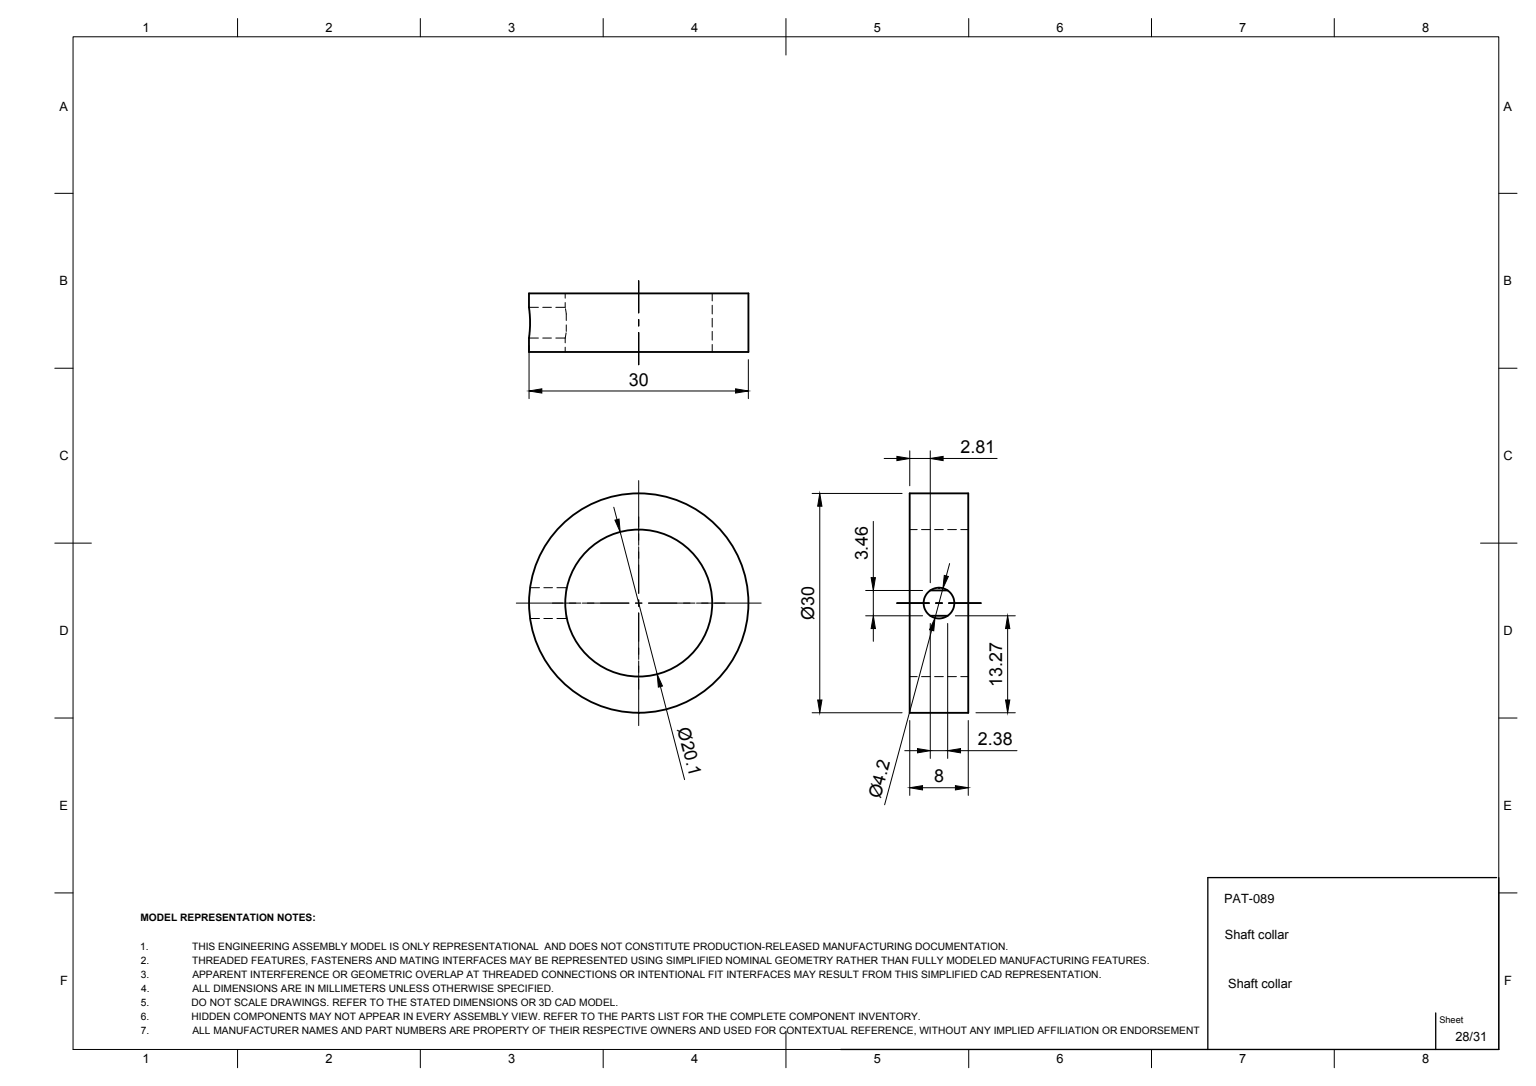
ISO-10303-21;
HEADER;
/* Generated by software containing ST-Developer
 * from STEP Tools, Inc. (www.steptools.com) 
 */

FILE_DESCRIPTION(
/* description */ ('Rotary union on bearing shaft'),
/* implementation_level */ '2;1');

FILE_NAME(
/* name */ 'Shaft collar.step',
/* time_stamp */ '2026-10-28T03:24:01-07:00',
/* author */ (''),
/* organization */ (''),
/* preprocessor_version */ 'ST-DEVELOPER v20.2',
/* originating_system */ 'Autodesk Translation Framework v15.17.0.0',
/* authorisation */ '');

FILE_SCHEMA (('AUTOMOTIVE_DESIGN { 1 0 10303 214 3 1 1 }'));
ENDSEC;

DATA;
#10=MECHANICAL_DESIGN_GEOMETRIC_PRESENTATION_REPRESENTATION('',(#341),#9448);
#255=B_SPLINE_CURVE_WITH_KNOTS('',3,(#8940,#8941,#8942,#8943,#8944,#8945,
#8946,#8947,#8948,#8949,#8950,#8951,#8952,#8953),.UNSPECIFIED.,.F.,.F.,
(4,2,2,2,2,2,4),(0.756005737987012,0.793568827564648,0.872922520054202,
0.952276212543757,1.03162990503331,1.11098359752287,1.1485466871005),
 .UNSPECIFIED.);
#256=B_SPLINE_CURVE_WITH_KNOTS('',3,(#8959,#8960,#8961,#8962,#8963,#8964,
#8965,#8966,#8967,#8968,#8969,#8970,#8971,#8972,#8973,#8974,#8975,#8976),
 .UNSPECIFIED.,.F.,.F.,(4,2,2,2,2,2,2,2,4),(0.,0.0792165807733632,0.158433161546726,
0.237648697074571,0.316864232602415,0.396079768130259,0.475295303658103,
0.554511884431466,0.63372846520483),.UNSPECIFIED.);
#257=B_SPLINE_CURVE_WITH_KNOTS('',3,(#8977,#8978,#8979,#8980,#8981,#8982,
#8983,#8984,#8985,#8986,#8987,#8988,#8989,#8990,#8991,#8992,#8993,#8994),
 .UNSPECIFIED.,.F.,.F.,(4,2,2,2,2,2,2,2,4),(0.63372846520483,0.712945045978192,
0.792161626751555,0.8713771622794,0.950592697807244,1.02980823333509,1.10902376886293,
1.1882403496363,1.26745693040966),.UNSPECIFIED.);
#258=B_SPLINE_CURVE_WITH_KNOTS('',3,(#8997,#8998,#8999,#9000,#9001,#9002,
#9003,#9004,#9005,#9006,#9007,#9008,#9009,#9010),.UNSPECIFIED.,.F.,.F.,
(4,2,2,2,2,2,4),(0.121154929624506,0.158718019202143,0.238071711691698,
0.317425404181252,0.396779096670807,0.476132789160362,0.513695878738),
 .UNSPECIFIED.);
#279=SHAPE_REPRESENTATION_RELATIONSHIP('SRR','None',#9581,#306);
#306=ADVANCED_BREP_SHAPE_REPRESENTATION('',(#374),#9441);
#341=STYLED_ITEM('',(#9778),#374);
#374=MANIFOLD_SOLID_BREP('Body1',#4898);
#464=FACE_BOUND('',#1264,.T.);
#465=FACE_BOUND('',#1266,.T.);
#466=FACE_BOUND('',#1268,.T.);
#467=FACE_BOUND('',#1270,.T.);
#604=PLANE('',#5662);
#605=PLANE('',#5667);
#606=PLANE('',#5674);
#607=PLANE('',#5675);
#877=FACE_OUTER_BOUND('',#1260,.T.);
#878=FACE_OUTER_BOUND('',#1261,.T.);
#879=FACE_OUTER_BOUND('',#1262,.T.);
#880=FACE_OUTER_BOUND('',#1263,.T.);
#881=FACE_OUTER_BOUND('',#1265,.T.);
#882=FACE_OUTER_BOUND('',#1267,.T.);
#883=FACE_OUTER_BOUND('',#1269,.T.);
#1260=EDGE_LOOP('',(#4151,#4152));
#1261=EDGE_LOOP('',(#4153,#4154,#4155,#4156,#4157,#4158,#4159,#4160,#4161));
#1262=EDGE_LOOP('',(#4162,#4163,#4164));
#1263=EDGE_LOOP('',(#4165,#4166,#4167,#4168));
#1264=EDGE_LOOP('',(#4169,#4170,#4171,#4172));
#1265=EDGE_LOOP('',(#4173,#4174,#4175,#4176));
#1266=EDGE_LOOP('',(#4177,#4178));
#1267=EDGE_LOOP('',(#4179));
#1268=EDGE_LOOP('',(#4180));
#1269=EDGE_LOOP('',(#4181));
#1270=EDGE_LOOP('',(#4182));
#1566=LINE('',#8936,#1886);
#1567=LINE('',#8957,#1887);
#1568=LINE('',#9012,#1888);
#1569=LINE('',#9017,#1889);
#1570=LINE('',#9023,#1890);
#1886=VECTOR('',#6951,1.);
#1887=VECTOR('',#6958,0.21);
#1888=VECTOR('',#6963,1.);
#1889=VECTOR('',#6968,1.005);
#1890=VECTOR('',#6975,1.5);
#2208=CIRCLE('',#5663,0.21);
#2209=CIRCLE('',#5665,0.21);
#2210=CIRCLE('',#5666,0.21);
#2211=CIRCLE('',#5669,1.005);
#2212=CIRCLE('',#5670,1.005);
#2213=CIRCLE('',#5672,1.5);
#2214=CIRCLE('',#5673,1.5);
#2554=VERTEX_POINT('',#8934);
#2555=VERTEX_POINT('',#8935);
#2556=VERTEX_POINT('',#8939);
#2557=VERTEX_POINT('',#8954);
#2558=VERTEX_POINT('',#8956);
#2559=VERTEX_POINT('',#8958);
#2560=VERTEX_POINT('',#8995);
#2561=VERTEX_POINT('',#9014);
#2562=VERTEX_POINT('',#9016);
#2563=VERTEX_POINT('',#9020);
#2564=VERTEX_POINT('',#9022);
#3103=EDGE_CURVE('',#2554,#2555,#1566,.T.);
#3104=EDGE_CURVE('',#2554,#2555,#2208,.T.);
#3105=EDGE_CURVE('',#2556,#2554,#255,.T.);
#3106=EDGE_CURVE('',#2557,#2556,#2209,.T.);
#3107=EDGE_CURVE('',#2557,#2558,#1567,.T.);
#3108=EDGE_CURVE('',#2559,#2558,#256,.T.);
#3109=EDGE_CURVE('',#2558,#2559,#257,.T.);
#3110=EDGE_CURVE('',#2560,#2557,#2210,.T.);
#3111=EDGE_CURVE('',#2555,#2560,#258,.T.);
#3112=EDGE_CURVE('',#2560,#2556,#1568,.T.);
#3113=EDGE_CURVE('',#2561,#2561,#2211,.T.);
#3114=EDGE_CURVE('',#2561,#2562,#1569,.T.);
#3115=EDGE_CURVE('',#2562,#2562,#2212,.T.);
#3116=EDGE_CURVE('',#2563,#2563,#2213,.T.);
#3117=EDGE_CURVE('',#2563,#2564,#1570,.T.);
#3118=EDGE_CURVE('',#2564,#2564,#2214,.T.);
#4151=ORIENTED_EDGE('',*,*,#3103,.F.);
#4152=ORIENTED_EDGE('',*,*,#3104,.T.);
#4153=ORIENTED_EDGE('',*,*,#3105,.F.);
#4154=ORIENTED_EDGE('',*,*,#3106,.F.);
#4155=ORIENTED_EDGE('',*,*,#3107,.T.);
#4156=ORIENTED_EDGE('',*,*,#3108,.F.);
#4157=ORIENTED_EDGE('',*,*,#3109,.F.);
#4158=ORIENTED_EDGE('',*,*,#3107,.F.);
#4159=ORIENTED_EDGE('',*,*,#3110,.F.);
#4160=ORIENTED_EDGE('',*,*,#3111,.F.);
#4161=ORIENTED_EDGE('',*,*,#3104,.F.);
#4162=ORIENTED_EDGE('',*,*,#3112,.F.);
#4163=ORIENTED_EDGE('',*,*,#3110,.T.);
#4164=ORIENTED_EDGE('',*,*,#3106,.T.);
#4165=ORIENTED_EDGE('',*,*,#3113,.F.);
#4166=ORIENTED_EDGE('',*,*,#3114,.T.);
#4167=ORIENTED_EDGE('',*,*,#3115,.T.);
#4168=ORIENTED_EDGE('',*,*,#3114,.F.);
#4169=ORIENTED_EDGE('',*,*,#3111,.T.);
#4170=ORIENTED_EDGE('',*,*,#3112,.T.);
#4171=ORIENTED_EDGE('',*,*,#3105,.T.);
#4172=ORIENTED_EDGE('',*,*,#3103,.T.);
#4173=ORIENTED_EDGE('',*,*,#3116,.F.);
#4174=ORIENTED_EDGE('',*,*,#3117,.T.);
#4175=ORIENTED_EDGE('',*,*,#3118,.T.);
#4176=ORIENTED_EDGE('',*,*,#3117,.F.);
#4177=ORIENTED_EDGE('',*,*,#3108,.T.);
#4178=ORIENTED_EDGE('',*,*,#3109,.T.);
#4179=ORIENTED_EDGE('',*,*,#3116,.T.);
#4180=ORIENTED_EDGE('',*,*,#3113,.T.);
#4181=ORIENTED_EDGE('',*,*,#3118,.F.);
#4182=ORIENTED_EDGE('',*,*,#3115,.F.);
#4551=CYLINDRICAL_SURFACE('',#5664,0.21);
#4552=CYLINDRICAL_SURFACE('',#5668,1.005);
#4553=CYLINDRICAL_SURFACE('',#5671,1.5);
#4790=ADVANCED_FACE('',(#877),#604,.T.);
#4791=ADVANCED_FACE('',(#878),#4551,.F.);
#4792=ADVANCED_FACE('',(#879),#605,.T.);
#4793=ADVANCED_FACE('',(#880,#464),#4552,.F.);
#4794=ADVANCED_FACE('',(#881,#465),#4553,.T.);
#4795=ADVANCED_FACE('',(#882,#466),#606,.T.);
#4796=ADVANCED_FACE('',(#883,#467),#607,.F.);
#4898=CLOSED_SHELL('',(#4790,#4791,#4792,#4793,#4794,#4795,#4796));
#5661=AXIS2_PLACEMENT_3D('',#8932,#6947,#6948);
#5662=AXIS2_PLACEMENT_3D('',#8933,#6949,#6950);
#5663=AXIS2_PLACEMENT_3D('',#8937,#6952,#6953);
#5664=AXIS2_PLACEMENT_3D('',#8938,#6954,#6955);
#5665=AXIS2_PLACEMENT_3D('',#8955,#6956,#6957);
#5666=AXIS2_PLACEMENT_3D('',#8996,#6959,#6960);
#5667=AXIS2_PLACEMENT_3D('',#9011,#6961,#6962);
#5668=AXIS2_PLACEMENT_3D('',#9013,#6964,#6965);
#5669=AXIS2_PLACEMENT_3D('',#9015,#6966,#6967);
#5670=AXIS2_PLACEMENT_3D('',#9018,#6969,#6970);
#5671=AXIS2_PLACEMENT_3D('',#9019,#6971,#6972);
#5672=AXIS2_PLACEMENT_3D('',#9021,#6973,#6974);
#5673=AXIS2_PLACEMENT_3D('',#9024,#6976,#6977);
#5674=AXIS2_PLACEMENT_3D('',#9025,#6978,#6979);
#5675=AXIS2_PLACEMENT_3D('',#9026,#6980,#6981);
#6947=DIRECTION('axis',(0.,0.,1.));
#6948=DIRECTION('refdir',(1.,0.,0.));
#6949=DIRECTION('center_axis',(0.,0.,1.));
#6950=DIRECTION('ref_axis',(1.,0.,0.));
#6951=DIRECTION('',(0.,1.,0.));
#6952=DIRECTION('center_axis',(0.,0.,1.));
#6953=DIRECTION('ref_axis',(1.,0.,0.));
#6954=DIRECTION('center_axis',(0.,0.,1.));
#6955=DIRECTION('ref_axis',(1.,0.,0.));
#6956=DIRECTION('center_axis',(0.,0.,1.));
#6957=DIRECTION('ref_axis',(1.,0.,0.));
#6958=DIRECTION('',(0.,0.,1.));
#6959=DIRECTION('center_axis',(0.,0.,1.));
#6960=DIRECTION('ref_axis',(1.,0.,0.));
#6961=DIRECTION('center_axis',(0.,0.,1.));
#6962=DIRECTION('ref_axis',(1.,0.,0.));
#6963=DIRECTION('',(0.,-1.,0.));
#6964=DIRECTION('center_axis',(0.,1.,0.));
#6965=DIRECTION('ref_axis',(1.,0.,0.));
#6966=DIRECTION('center_axis',(0.,-1.,0.));
#6967=DIRECTION('ref_axis',(1.,0.,0.));
#6968=DIRECTION('',(0.,-1.,0.));
#6969=DIRECTION('center_axis',(0.,-1.,0.));
#6970=DIRECTION('ref_axis',(1.,0.,0.));
#6971=DIRECTION('center_axis',(0.,1.,0.));
#6972=DIRECTION('ref_axis',(1.,0.,0.));
#6973=DIRECTION('center_axis',(0.,1.,0.));
#6974=DIRECTION('ref_axis',(1.,0.,0.));
#6975=DIRECTION('',(0.,-1.,0.));
#6976=DIRECTION('center_axis',(0.,1.,0.));
#6977=DIRECTION('ref_axis',(1.,0.,0.));
#6978=DIRECTION('center_axis',(0.,1.,0.));
#6979=DIRECTION('ref_axis',(1.,0.,0.));
#6980=DIRECTION('center_axis',(0.,1.,0.));
#6981=DIRECTION('ref_axis',(1.,0.,0.));
#8932=CARTESIAN_POINT('',(0.,0.,0.));
#8933=CARTESIAN_POINT('Origin',(0.,6.8,5.49));
#8934=CARTESIAN_POINT('',(0.172988438920061,6.68094119100209,5.49));
#8935=CARTESIAN_POINT('',(0.172988438920061,6.91905880899791,5.49));
#8936=CARTESIAN_POINT('',(0.172988438920061,6.4,5.49));
#8937=CARTESIAN_POINT('Origin',(0.,6.8,5.49));
#8938=CARTESIAN_POINT('Origin',(0.,6.8,5.49));
#8939=CARTESIAN_POINT('',(-0.172988438920061,6.68094119100209,5.49));
#8940=CARTESIAN_POINT('Ctrl Pts',(-0.172988438920061,6.68094119100209,5.49));
#8941=CARTESIAN_POINT('Ctrl Pts',(-0.165594865311318,6.67019857760471,5.49129192197638));
#8942=CARTESIAN_POINT('Ctrl Pts',(-0.157297138725608,6.66031229062726,5.49265394943905));
#8943=CARTESIAN_POINT('Ctrl Pts',(-0.129892073845076,6.63290722574673,5.4967480843909));
#8944=CARTESIAN_POINT('Ctrl Pts',(-0.106330167759285,6.61675794366705,5.49969589327638));
#8945=CARTESIAN_POINT('Ctrl Pts',(-0.0546129046324107,6.59530220603509,
5.50385029472357));
#8946=CARTESIAN_POINT('Ctrl Pts',(-0.0264512308298516,6.59,5.505));
#8947=CARTESIAN_POINT('Ctrl Pts',(0.0264512308298515,6.59,5.505));
#8948=CARTESIAN_POINT('Ctrl Pts',(0.0546129046324106,6.59530220603509,5.50385029472357));
#8949=CARTESIAN_POINT('Ctrl Pts',(0.106330167759285,6.61675794366705,5.49969589327638));
#8950=CARTESIAN_POINT('Ctrl Pts',(0.129892073845076,6.63290722574673,5.4967480843909));
#8951=CARTESIAN_POINT('Ctrl Pts',(0.157297138725608,6.66031229062726,5.49265394943905));
#8952=CARTESIAN_POINT('Ctrl Pts',(0.165594865311318,6.67019857760471,5.49129192197638));
#8953=CARTESIAN_POINT('Ctrl Pts',(0.172988438920061,6.68094119100209,5.49));
#8954=CARTESIAN_POINT('',(-0.21,6.8,5.49));
#8955=CARTESIAN_POINT('Origin',(0.,6.8,5.49));
#8956=CARTESIAN_POINT('',(-0.21,6.8,5.98522725533839));
#8957=CARTESIAN_POINT('',(-0.21,6.8,5.49));
#8958=CARTESIAN_POINT('',(0.21,6.8,5.98522725533839));
#8959=CARTESIAN_POINT('Ctrl Pts',(0.21,6.8,5.98522725533839));
#8960=CARTESIAN_POINT('Ctrl Pts',(0.21,6.77359447307555,5.98522725533839));
#8961=CARTESIAN_POINT('Ctrl Pts',(0.204715737269596,6.74545292590929,5.98600415954412));
#8962=CARTESIAN_POINT('Ctrl Pts',(0.183273763036331,6.69372373109487,5.98880073282317));
#8963=CARTESIAN_POINT('Ctrl Pts',(0.167117923970394,6.67013307587204,5.99077897157582));
#8964=CARTESIAN_POINT('Ctrl Pts',(0.129867169887369,6.63288232178902,5.99448481141327));
#8965=CARTESIAN_POINT('Ctrl Pts',(0.106276408305765,6.61672628999865,5.99645455657129));
#8966=CARTESIAN_POINT('Ctrl Pts',(0.0545468514059003,6.59528417517378,5.99923165515646));
#8967=CARTESIAN_POINT('Ctrl Pts',(0.0264051785092814,6.59,6.));
#8968=CARTESIAN_POINT('Ctrl Pts',(-0.0264051785092814,6.59,6.));
#8969=CARTESIAN_POINT('Ctrl Pts',(-0.0545468514059002,6.59528417517378,
5.99923165515646));
#8970=CARTESIAN_POINT('Ctrl Pts',(-0.106276408305765,6.61672628999865,5.99645455657129));
#8971=CARTESIAN_POINT('Ctrl Pts',(-0.129867169887369,6.63288232178902,5.99448481141327));
#8972=CARTESIAN_POINT('Ctrl Pts',(-0.167117923970394,6.67013307587204,5.99077897157582));
#8973=CARTESIAN_POINT('Ctrl Pts',(-0.183273763036331,6.69372373109487,5.98880073282317));
#8974=CARTESIAN_POINT('Ctrl Pts',(-0.204715737269596,6.74545292590929,5.98600415954412));
#8975=CARTESIAN_POINT('Ctrl Pts',(-0.21,6.77359447307555,5.98522725533839));
#8976=CARTESIAN_POINT('Ctrl Pts',(-0.21,6.8,5.98522725533839));
#8977=CARTESIAN_POINT('Ctrl Pts',(-0.21,6.8,5.98522725533839));
#8978=CARTESIAN_POINT('Ctrl Pts',(-0.21,6.82640552692445,5.98522725533839));
#8979=CARTESIAN_POINT('Ctrl Pts',(-0.204715737269596,6.85454707409071,5.98600415954412));
#8980=CARTESIAN_POINT('Ctrl Pts',(-0.183273763036331,6.90627626890513,5.98880073282317));
#8981=CARTESIAN_POINT('Ctrl Pts',(-0.167117923970394,6.92986692412796,5.99077897157582));
#8982=CARTESIAN_POINT('Ctrl Pts',(-0.129867169887369,6.96711767821098,5.99448481141327));
#8983=CARTESIAN_POINT('Ctrl Pts',(-0.106276408305765,6.98327371000135,5.99645455657129));
#8984=CARTESIAN_POINT('Ctrl Pts',(-0.0545468514059003,7.00471582482622,
5.99923165515646));
#8985=CARTESIAN_POINT('Ctrl Pts',(-0.0264051785092815,7.01,6.));
#8986=CARTESIAN_POINT('Ctrl Pts',(0.0264051785092814,7.01,6.));
#8987=CARTESIAN_POINT('Ctrl Pts',(0.0545468514058999,7.00471582482622,5.99923165515646));
#8988=CARTESIAN_POINT('Ctrl Pts',(0.106276408305765,6.98327371000135,5.99645455657129));
#8989=CARTESIAN_POINT('Ctrl Pts',(0.129867169887369,6.96711767821098,5.99448481141327));
#8990=CARTESIAN_POINT('Ctrl Pts',(0.167117923970393,6.92986692412796,5.99077897157582));
#8991=CARTESIAN_POINT('Ctrl Pts',(0.183273763036332,6.90627626890513,5.98880073282317));
#8992=CARTESIAN_POINT('Ctrl Pts',(0.204715737269596,6.85454707409071,5.98600415954412));
#8993=CARTESIAN_POINT('Ctrl Pts',(0.21,6.82640552692445,5.98522725533839));
#8994=CARTESIAN_POINT('Ctrl Pts',(0.21,6.8,5.98522725533839));
#8995=CARTESIAN_POINT('',(-0.172988438920061,6.91905880899791,5.49));
#8996=CARTESIAN_POINT('Origin',(0.,6.8,5.49));
#8997=CARTESIAN_POINT('Ctrl Pts',(0.172988438920062,6.91905880899791,5.49));
#8998=CARTESIAN_POINT('Ctrl Pts',(0.165594865311319,6.92980142239529,5.49129192197638));
#8999=CARTESIAN_POINT('Ctrl Pts',(0.157297138725609,6.93968770937274,5.49265394943905));
#9000=CARTESIAN_POINT('Ctrl Pts',(0.129892073845076,6.96709277425327,5.4967480843909));
#9001=CARTESIAN_POINT('Ctrl Pts',(0.106330167759285,6.98324205633295,5.49969589327638));
#9002=CARTESIAN_POINT('Ctrl Pts',(0.0546129046324107,7.00469779396491,5.50385029472357));
#9003=CARTESIAN_POINT('Ctrl Pts',(0.0264512308298516,7.01,5.505));
#9004=CARTESIAN_POINT('Ctrl Pts',(-0.0264512308298515,7.01,5.505));
#9005=CARTESIAN_POINT('Ctrl Pts',(-0.0546129046324097,7.00469779396491,
5.50385029472357));
#9006=CARTESIAN_POINT('Ctrl Pts',(-0.106330167759284,6.98324205633295,5.49969589327638));
#9007=CARTESIAN_POINT('Ctrl Pts',(-0.129892073845076,6.96709277425327,5.4967480843909));
#9008=CARTESIAN_POINT('Ctrl Pts',(-0.157297138725609,6.93968770937274,5.49265394943905));
#9009=CARTESIAN_POINT('Ctrl Pts',(-0.165594865311318,6.92980142239529,5.49129192197638));
#9010=CARTESIAN_POINT('Ctrl Pts',(-0.172988438920061,6.91905880899791,5.49));
#9011=CARTESIAN_POINT('Origin',(0.,6.8,5.49));
#9012=CARTESIAN_POINT('',(-0.172988438920061,6.4,5.49));
#9013=CARTESIAN_POINT('Origin',(0.,6.4,4.5));
#9014=CARTESIAN_POINT('',(-1.005,7.2,4.5));
#9015=CARTESIAN_POINT('Origin',(0.,7.2,4.5));
#9016=CARTESIAN_POINT('',(-1.005,6.4,4.5));
#9017=CARTESIAN_POINT('',(-1.005,6.4,4.5));
#9018=CARTESIAN_POINT('Origin',(0.,6.4,4.5));
#9019=CARTESIAN_POINT('Origin',(0.,6.4,4.5));
#9020=CARTESIAN_POINT('',(-1.5,7.2,4.5));
#9021=CARTESIAN_POINT('Origin',(0.,7.2,4.5));
#9022=CARTESIAN_POINT('',(-1.5,6.4,4.5));
#9023=CARTESIAN_POINT('',(-1.5,6.4,4.5));
#9024=CARTESIAN_POINT('Origin',(0.,6.4,4.5));
#9025=CARTESIAN_POINT('Origin',(0.,7.2,4.5));
#9026=CARTESIAN_POINT('Origin',(0.,6.4,4.5));
#9409=UNCERTAINTY_MEASURE_WITH_UNIT(LENGTH_MEASURE(0.001),#9449,
'DISTANCE_ACCURACY_VALUE',
'Maximum model space distance between geometric entities at asserted c
onnectivities');
#9416=UNCERTAINTY_MEASURE_WITH_UNIT(LENGTH_MEASURE(0.001),#9449,
'DISTANCE_ACCURACY_VALUE',
'Maximum model space distance between geometric entities at asserted c
onnectivities');
#9441=(
GEOMETRIC_REPRESENTATION_CONTEXT(3)
GLOBAL_UNCERTAINTY_ASSIGNED_CONTEXT((#9409))
GLOBAL_UNIT_ASSIGNED_CONTEXT((#9449,#9451,#9452))
REPRESENTATION_CONTEXT('','3D')
);
#9448=(
GEOMETRIC_REPRESENTATION_CONTEXT(3)
GLOBAL_UNCERTAINTY_ASSIGNED_CONTEXT((#9416))
GLOBAL_UNIT_ASSIGNED_CONTEXT((#9449,#9451,#9452))
REPRESENTATION_CONTEXT('','3D')
);
#9449=(
LENGTH_UNIT()
NAMED_UNIT(*)
SI_UNIT(.CENTI.,.METRE.)
);
#9451=(
NAMED_UNIT(*)
PLANE_ANGLE_UNIT()
SI_UNIT($,.RADIAN.)
);
#9452=(
NAMED_UNIT(*)
SI_UNIT($,.STERADIAN.)
SOLID_ANGLE_UNIT()
);
#9477=SHAPE_DEFINITION_REPRESENTATION(#9513,#9581);
#9513=PRODUCT_DEFINITION_SHAPE('',$,#9613);
#9581=SHAPE_REPRESENTATION('',(#5661),#9441);
#9588=PRODUCT_DEFINITION_CONTEXT('part definition',#9683,'design');
#9613=PRODUCT_DEFINITION('Shaft collar','Shaft collar',#9644,#9588);
#9644=PRODUCT_DEFINITION_FORMATION('',$,#9709);
#9683=APPLICATION_CONTEXT(
'Core Data for Automotive Mechanical Design Process');
#9684=PRODUCT_CONTEXT('part definition',#9683,'mechanical');
#9709=PRODUCT('Shaft collar','Shaft collar','Shaft collar',(#9684));
#9772=COLOUR_RGB('Grey',0.48,0.52,0.57);
#9773=FILL_AREA_STYLE_COLOUR('',#9772);
#9774=FILL_AREA_STYLE('',(#9773));
#9775=SURFACE_STYLE_FILL_AREA(#9774);
#9776=SURFACE_SIDE_STYLE('',(#9775));
#9777=SURFACE_STYLE_USAGE(.BOTH.,#9776);
#9778=PRESENTATION_STYLE_ASSIGNMENT((#9777));
ENDSEC;
END-ISO-10303-21;
